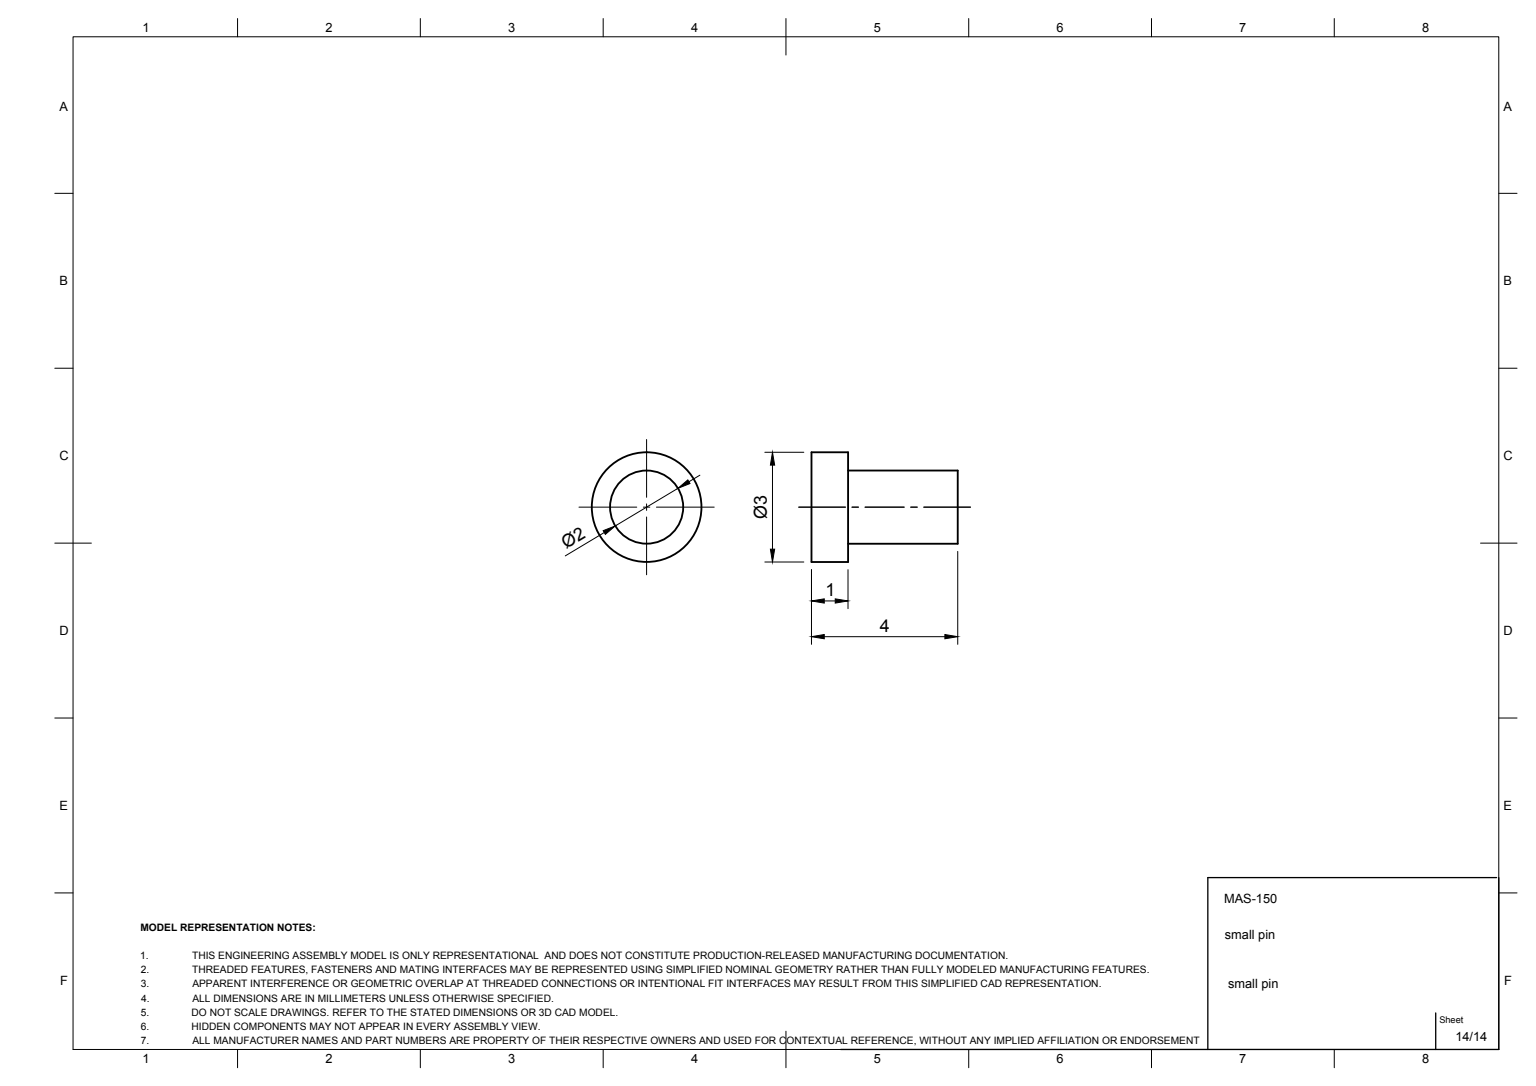
ISO-10303-21;
HEADER;
/* Generated by software containing ST-Developer
 * from STEP Tools, Inc. (www.steptools.com) 
 */

FILE_DESCRIPTION(
/* description */ ('STEP AP203'),
/* implementation_level */ '2;1');

FILE_NAME(
/* name */ 'small pin.step',
/* time_stamp */ '2026-11-08T21:40:52-08:00',
/* author */ (''),
/* organization */ (''),
/* preprocessor_version */ 'ST-DEVELOPER v20.2',
/* originating_system */ 'Autodesk Translation Framework v15.17.0.0',
/* authorisation */ '');

FILE_SCHEMA (('AUTOMOTIVE_DESIGN { 1 0 10303 214 3 1 1 }'));
ENDSEC;

DATA;
#10=MECHANICAL_DESIGN_GEOMETRIC_PRESENTATION_REPRESENTATION('',(#188),#12137);
#166=SHAPE_REPRESENTATION_RELATIONSHIP('SRR','None',#12190,#177);
#177=ADVANCED_BREP_SHAPE_REPRESENTATION('',(#199),#12131);
#188=STYLED_ITEM('',(#12253),#199);
#199=MANIFOLD_SOLID_BREP('Body1',#1833);
#219=FACE_BOUND('',#672,.T.);
#254=PLANE('',#2043);
#255=PLANE('',#2044);
#256=PLANE('',#2045);
#336=LINE('',#5258,#430);
#337=LINE('',#5264,#431);
#430=VECTOR('',#2376,1.);
#431=VECTOR('',#2383,1.5);
#475=CYLINDRICAL_SURFACE('',#2037,1.);
#476=CYLINDRICAL_SURFACE('',#2040,1.5);
#545=FACE_OUTER_BOUND('',#669,.T.);
#546=FACE_OUTER_BOUND('',#670,.T.);
#547=FACE_OUTER_BOUND('',#671,.T.);
#548=FACE_OUTER_BOUND('',#673,.T.);
#549=FACE_OUTER_BOUND('',#674,.T.);
#669=EDGE_LOOP('',(#1485,#1486,#1487,#1488));
#670=EDGE_LOOP('',(#1489,#1490,#1491,#1492));
#671=EDGE_LOOP('',(#1493));
#672=EDGE_LOOP('',(#1494));
#673=EDGE_LOOP('',(#1495));
#674=EDGE_LOOP('',(#1496));
#768=CIRCLE('',#2038,1.);
#769=CIRCLE('',#2039,1.);
#770=CIRCLE('',#2041,1.5);
#771=CIRCLE('',#2042,1.5);
#910=VERTEX_POINT('',#5255);
#911=VERTEX_POINT('',#5257);
#912=VERTEX_POINT('',#5261);
#913=VERTEX_POINT('',#5263);
#1112=EDGE_CURVE('',#910,#910,#768,.T.);
#1113=EDGE_CURVE('',#910,#911,#336,.T.);
#1114=EDGE_CURVE('',#911,#911,#769,.T.);
#1115=EDGE_CURVE('',#912,#912,#770,.T.);
#1116=EDGE_CURVE('',#912,#913,#337,.T.);
#1117=EDGE_CURVE('',#913,#913,#771,.T.);
#1485=ORIENTED_EDGE('',*,*,#1112,.T.);
#1486=ORIENTED_EDGE('',*,*,#1113,.T.);
#1487=ORIENTED_EDGE('',*,*,#1114,.F.);
#1488=ORIENTED_EDGE('',*,*,#1113,.F.);
#1489=ORIENTED_EDGE('',*,*,#1115,.T.);
#1490=ORIENTED_EDGE('',*,*,#1116,.T.);
#1491=ORIENTED_EDGE('',*,*,#1117,.F.);
#1492=ORIENTED_EDGE('',*,*,#1116,.F.);
#1493=ORIENTED_EDGE('',*,*,#1117,.T.);
#1494=ORIENTED_EDGE('',*,*,#1112,.F.);
#1495=ORIENTED_EDGE('',*,*,#1115,.F.);
#1496=ORIENTED_EDGE('',*,*,#1114,.T.);
#1773=ADVANCED_FACE('',(#545),#475,.T.);
#1774=ADVANCED_FACE('',(#546),#476,.T.);
#1775=ADVANCED_FACE('',(#547,#219),#254,.T.);
#1776=ADVANCED_FACE('',(#548),#255,.F.);
#1777=ADVANCED_FACE('',(#549),#256,.T.);
#1833=CLOSED_SHELL('',(#1773,#1774,#1775,#1776,#1777));
#2036=AXIS2_PLACEMENT_3D('',#5253,#2370,#2371);
#2037=AXIS2_PLACEMENT_3D('',#5254,#2372,#2373);
#2038=AXIS2_PLACEMENT_3D('',#5256,#2374,#2375);
#2039=AXIS2_PLACEMENT_3D('',#5259,#2377,#2378);
#2040=AXIS2_PLACEMENT_3D('',#5260,#2379,#2380);
#2041=AXIS2_PLACEMENT_3D('',#5262,#2381,#2382);
#2042=AXIS2_PLACEMENT_3D('',#5265,#2384,#2385);
#2043=AXIS2_PLACEMENT_3D('',#5266,#2386,#2387);
#2044=AXIS2_PLACEMENT_3D('',#5267,#2388,#2389);
#2045=AXIS2_PLACEMENT_3D('',#5268,#2390,#2391);
#2370=DIRECTION('axis',(0.,0.,1.));
#2371=DIRECTION('refdir',(1.,0.,0.));
#2372=DIRECTION('center_axis',(-1.,0.,0.));
#2373=DIRECTION('ref_axis',(0.,0.,1.));
#2374=DIRECTION('center_axis',(1.,0.,0.));
#2375=DIRECTION('ref_axis',(0.,0.,-1.));
#2376=DIRECTION('',(1.,0.,0.));
#2377=DIRECTION('center_axis',(1.,0.,0.));
#2378=DIRECTION('ref_axis',(0.,0.,-1.));
#2379=DIRECTION('center_axis',(-1.,0.,0.));
#2380=DIRECTION('ref_axis',(0.,0.,1.));
#2381=DIRECTION('center_axis',(1.,0.,0.));
#2382=DIRECTION('ref_axis',(0.,0.,-1.));
#2383=DIRECTION('',(1.,0.,0.));
#2384=DIRECTION('center_axis',(1.,0.,0.));
#2385=DIRECTION('ref_axis',(0.,0.,-1.));
#2386=DIRECTION('center_axis',(1.,0.,0.));
#2387=DIRECTION('ref_axis',(0.,0.,-1.));
#2388=DIRECTION('center_axis',(1.,0.,0.));
#2389=DIRECTION('ref_axis',(0.,0.,-1.));
#2390=DIRECTION('center_axis',(1.,0.,0.));
#2391=DIRECTION('ref_axis',(0.,0.,-1.));
#5253=CARTESIAN_POINT('',(0.,0.,0.));
#5254=CARTESIAN_POINT('Origin',(4.,0.,0.));
#5255=CARTESIAN_POINT('',(1.,-1.22464679914735E-16,-1.));
#5256=CARTESIAN_POINT('Origin',(1.,0.,0.));
#5257=CARTESIAN_POINT('',(4.,-1.22464679914735E-16,-1.));
#5258=CARTESIAN_POINT('',(4.,-1.22464679914735E-16,-1.));
#5259=CARTESIAN_POINT('Origin',(4.,0.,0.));
#5260=CARTESIAN_POINT('Origin',(1.,0.,0.));
#5261=CARTESIAN_POINT('',(0.,-1.83697019872103E-16,-1.5));
#5262=CARTESIAN_POINT('Origin',(0.,0.,0.));
#5263=CARTESIAN_POINT('',(1.,-1.83697019872103E-16,-1.5));
#5264=CARTESIAN_POINT('',(1.,-1.83697019872103E-16,-1.5));
#5265=CARTESIAN_POINT('Origin',(1.,0.,0.));
#5266=CARTESIAN_POINT('Origin',(1.,0.,0.));
#5267=CARTESIAN_POINT('Origin',(0.,0.,0.));
#5268=CARTESIAN_POINT('Origin',(4.,0.,0.));
#12117=UNCERTAINTY_MEASURE_WITH_UNIT(LENGTH_MEASURE(0.01),#12138,
'DISTANCE_ACCURACY_VALUE',
'Maximum model space distance between geometric entities at asserted c
onnectivities');
#12123=UNCERTAINTY_MEASURE_WITH_UNIT(LENGTH_MEASURE(0.01),#12138,
'DISTANCE_ACCURACY_VALUE',
'Maximum model space distance between geometric entities at asserted c
onnectivities');
#12131=(
GEOMETRIC_REPRESENTATION_CONTEXT(3)
GLOBAL_UNCERTAINTY_ASSIGNED_CONTEXT((#12117))
GLOBAL_UNIT_ASSIGNED_CONTEXT((#12138,#12140,#12141))
REPRESENTATION_CONTEXT('','3D')
);
#12137=(
GEOMETRIC_REPRESENTATION_CONTEXT(3)
GLOBAL_UNCERTAINTY_ASSIGNED_CONTEXT((#12123))
GLOBAL_UNIT_ASSIGNED_CONTEXT((#12138,#12140,#12141))
REPRESENTATION_CONTEXT('','3D')
);
#12138=(
LENGTH_UNIT()
NAMED_UNIT(*)
SI_UNIT(.MILLI.,.METRE.)
);
#12140=(
NAMED_UNIT(*)
PLANE_ANGLE_UNIT()
SI_UNIT($,.RADIAN.)
);
#12141=(
NAMED_UNIT(*)
SI_UNIT($,.STERADIAN.)
SOLID_ANGLE_UNIT()
);
#12149=SHAPE_DEFINITION_REPRESENTATION(#12162,#12190);
#12162=PRODUCT_DEFINITION_SHAPE('',$,#12204);
#12190=SHAPE_REPRESENTATION('',(#2036),#12131);
#12196=PRODUCT_DEFINITION_CONTEXT('part definition',#12237,'design');
#12204=PRODUCT_DEFINITION('small pin','small pin',#12217,#12196);
#12217=PRODUCT_DEFINITION_FORMATION('',$,#12246);
#12237=APPLICATION_CONTEXT(
'Core Data for Automotive Mechanical Design Process');
#12238=PRODUCT_CONTEXT('part definition',#12237,'mechanical');
#12246=PRODUCT('small pin','small pin',$,(#12238));
#12253=PRESENTATION_STYLE_ASSIGNMENT((#12255));
#12255=SURFACE_STYLE_USAGE(.BOTH.,#12257);
#12257=SURFACE_SIDE_STYLE('',(#12259));
#12259=SURFACE_STYLE_FILL_AREA(#12261);
#12261=FILL_AREA_STYLE('Opaque(23,69,131)',(#12263));
#12263=FILL_AREA_STYLE_COLOUR('Opaque(23,69,131)',#12265);
#12265=COLOUR_RGB('Opaque(23,69,131)',0.0901960784313725,0.270588235294118,
0.513725490196078);
ENDSEC;
END-ISO-10303-21;
